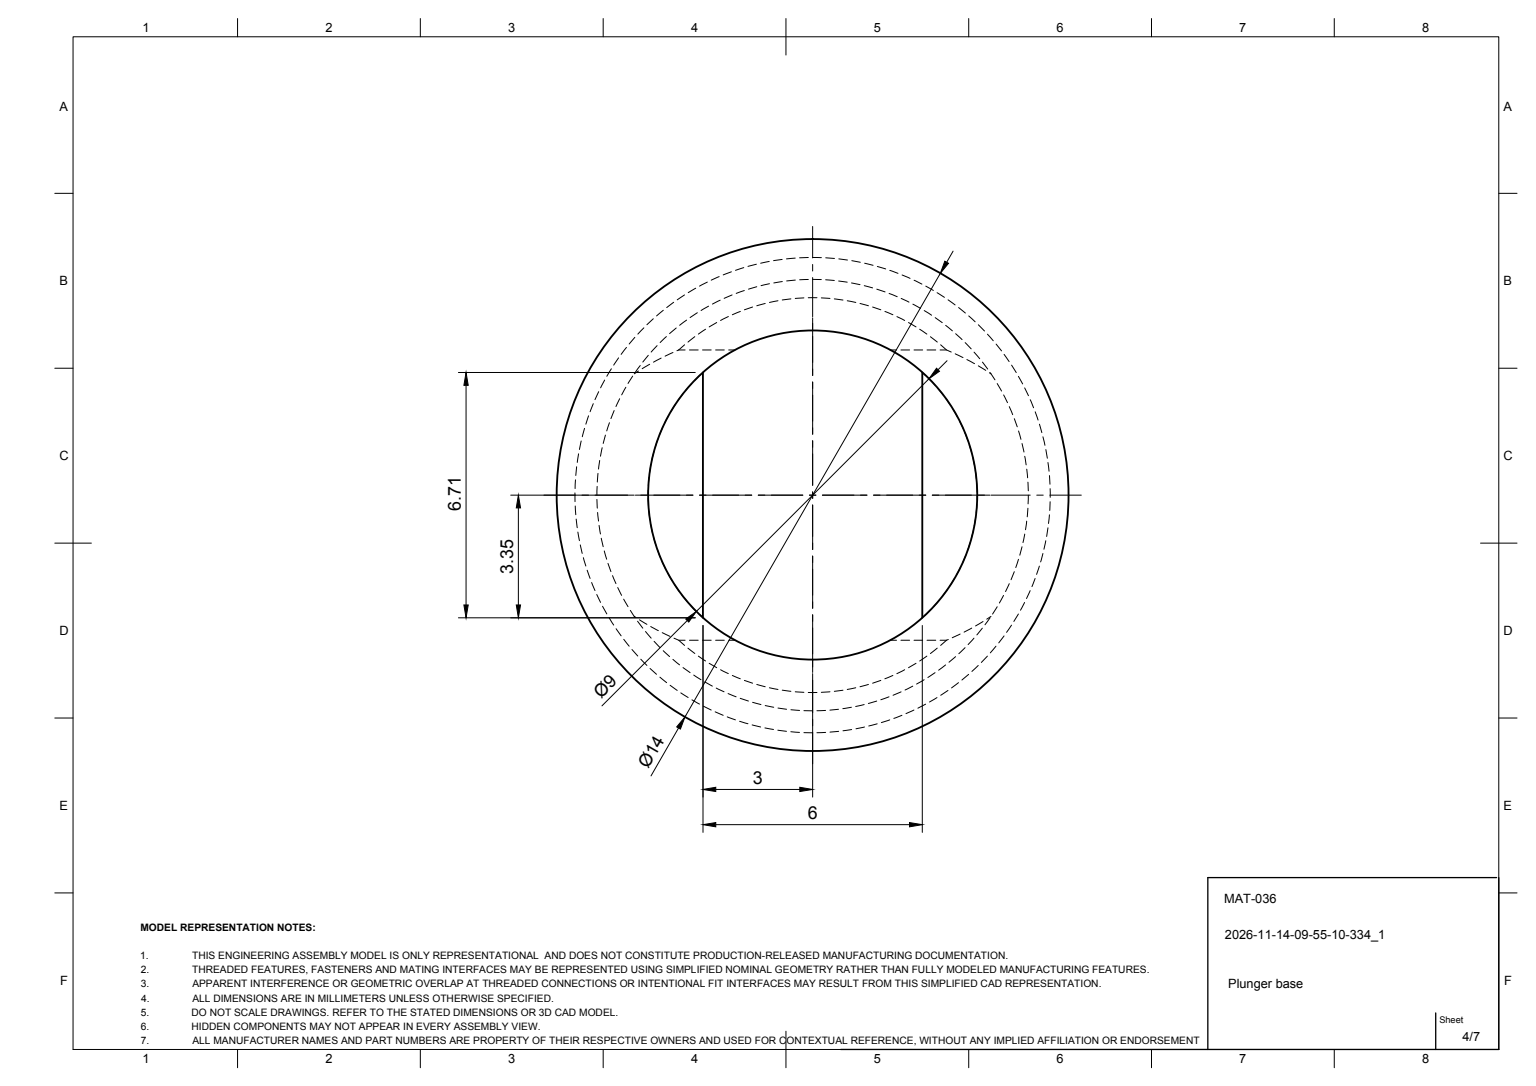
ISO-10303-21;
HEADER;
/* Generated by software containing ST-Developer
 * from STEP Tools, Inc. (www.steptools.com) 
 */

FILE_DESCRIPTION(
/* description */ (''),
/* implementation_level */ '2;1');

FILE_NAME(
/* name */ 'Plunger base.step',
/* time_stamp */ '2026-11-14T09:55:16-08:00',
/* author */ (''),
/* organization */ (''),
/* preprocessor_version */ 'ST-DEVELOPER v20.2',
/* originating_system */ 'Autodesk Translation Framework v15.17.0.0',
/* authorisation */ '');

FILE_SCHEMA (('AUTOMOTIVE_DESIGN { 1 0 10303 214 3 1 1 }'));
ENDSEC;

DATA;
#10=MECHANICAL_DESIGN_GEOMETRIC_PRESENTATION_REPRESENTATION('',(#57,#58,#59),#170250);
#40=OPEN_SHELL('',(#71352));
#41=OPEN_SHELL('',(#71353));
#42=SHELL_BASED_SURFACE_MODEL('Body2',(#40));
#43=SHELL_BASED_SURFACE_MODEL('Body3',(#41));
#45=SHAPE_REPRESENTATION_RELATIONSHIP('SRR','None',#170277,#51);
#51=ADVANCED_BREP_SHAPE_REPRESENTATION('',(#65),#170245);
#57=STYLED_ITEM('',(#170314),#65);
#58=STYLED_ITEM('',(#170314),#42);
#59=STYLED_ITEM('',(#170314),#43);
#65=MANIFOLD_SOLID_BREP('Body1',#71399);
#74=FACE_BOUND('',#15862,.T.);
#75=FACE_BOUND('',#15864,.T.);
#90=PLANE('',#77665);
#91=PLANE('',#77666);
#92=PLANE('',#77667);
#93=PLANE('',#77670);
#94=PLANE('',#77672);
#95=PLANE('',#77673);
#96=PLANE('',#77674);
#97=PLANE('',#77675);
#5361=CYLINDRICAL_SURFACE('',#77642,7.);
#5362=CYLINDRICAL_SURFACE('',#77645,4.5);
#5363=CYLINDRICAL_SURFACE('',#77652,6.5);
#5364=CYLINDRICAL_SURFACE('',#77656,5.99999999999999);
#5365=CYLINDRICAL_SURFACE('',#77663,5.9);
#5366=CYLINDRICAL_SURFACE('',#77669,5.99999999999999);
#5367=CYLINDRICAL_SURFACE('',#77677,6.);
#5368=CYLINDRICAL_SURFACE('',#77679,6.);
#10585=FACE_OUTER_BOUND('',#15854,.T.);
#10586=FACE_OUTER_BOUND('',#15855,.T.);
#10587=FACE_OUTER_BOUND('',#15856,.T.);
#10588=FACE_OUTER_BOUND('',#15857,.T.);
#10589=FACE_OUTER_BOUND('',#15858,.T.);
#10590=FACE_OUTER_BOUND('',#15859,.T.);
#10591=FACE_OUTER_BOUND('',#15860,.T.);
#10592=FACE_OUTER_BOUND('',#15861,.T.);
#10593=FACE_OUTER_BOUND('',#15863,.T.);
#10594=FACE_OUTER_BOUND('',#15865,.T.);
#10595=FACE_OUTER_BOUND('',#15866,.T.);
#10596=FACE_OUTER_BOUND('',#15867,.T.);
#10597=FACE_OUTER_BOUND('',#15868,.T.);
#10598=FACE_OUTER_BOUND('',#15869,.T.);
#10599=FACE_OUTER_BOUND('',#15870,.T.);
#10600=FACE_OUTER_BOUND('',#15871,.T.);
#10601=FACE_OUTER_BOUND('',#15872,.T.);
#10602=FACE_OUTER_BOUND('',#15873,.T.);
#10603=FACE_OUTER_BOUND('',#15874,.T.);
#15854=EDGE_LOOP('',(#65684,#65685,#65686,#65687));
#15855=EDGE_LOOP('',(#65688,#65689,#65690,#65691,#65692,#65693,#65694,#65695,
#65696,#65697,#65698,#65699,#65700,#65701,#65702,#65703));
#15856=EDGE_LOOP('',(#65704,#65705,#65706,#65707,#65708));
#15857=EDGE_LOOP('',(#65709,#65710,#65711,#65712,#65713,#65714,#65715,#65716));
#15858=EDGE_LOOP('',(#65717,#65718,#65719,#65720,#65721));
#15859=EDGE_LOOP('',(#65722,#65723,#65724,#65725));
#15860=EDGE_LOOP('',(#65726,#65727,#65728,#65729,#65730,#65731,#65732,#65733));
#15861=EDGE_LOOP('',(#65734));
#15862=EDGE_LOOP('',(#65735));
#15863=EDGE_LOOP('',(#65736));
#15864=EDGE_LOOP('',(#65737));
#15865=EDGE_LOOP('',(#65738,#65739,#65740,#65741));
#15866=EDGE_LOOP('',(#65742,#65743,#65744,#65745,#65746,#65747,#65748,#65749,
#65750));
#15867=EDGE_LOOP('',(#65751,#65752,#65753,#65754));
#15868=EDGE_LOOP('',(#65755,#65756,#65757,#65758));
#15869=EDGE_LOOP('',(#65759,#65760));
#15870=EDGE_LOOP('',(#65761,#65762,#65763));
#15871=EDGE_LOOP('',(#65764,#65765,#65766,#65767));
#15872=EDGE_LOOP('',(#65768,#65769,#65770,#65771));
#15873=EDGE_LOOP('',(#65772,#65773,#65774));
#15874=EDGE_LOOP('',(#65775,#65776,#65777));
#20991=CIRCLE('',#77643,7.);
#20992=CIRCLE('',#77644,7.);
#20993=CIRCLE('',#77646,4.5);
#20994=CIRCLE('',#77647,4.5);
#20995=CIRCLE('',#77648,4.5);
#20996=CIRCLE('',#77649,4.5);
#20997=CIRCLE('',#77650,4.5);
#20998=CIRCLE('',#77651,4.5);
#20999=CIRCLE('',#77653,6.5);
#21000=CIRCLE('',#77654,6.5);
#21001=CIRCLE('',#77655,6.5);
#21002=CIRCLE('',#77657,5.99999999999999);
#21003=CIRCLE('',#77659,5.9);
#21004=CIRCLE('',#77661,5.39999999999997);
#21005=CIRCLE('',#77662,5.9);
#21006=CIRCLE('',#77664,5.9);
#21007=CIRCLE('',#77668,5.99999999999999);
#21008=CIRCLE('',#77671,5.4);
#21009=CIRCLE('',#77678,6.);
#21010=CIRCLE('',#77680,6.);
#24303=B_SPLINE_CURVE_WITH_KNOTS('',3,(#168059,#168060,#168061,#168062),
 .UNSPECIFIED.,.F.,.F.,(4,4),(1.09971404256795,1.21244876000028),
 .UNSPECIFIED.);
#24304=B_SPLINE_CURVE_WITH_KNOTS('',3,(#168066,#168067,#168068,#168069),
 .UNSPECIFIED.,.F.,.F.,(4,4),(1.65787808514986,1.77061280261397),
 .UNSPECIFIED.);
#24305=B_SPLINE_CURVE_WITH_KNOTS('',3,(#168082,#168083,#168084,#168085),
 .UNSPECIFIED.,.F.,.F.,(4,4),(2.53487746522254,2.64761218276488),
 .UNSPECIFIED.);
#24306=B_SPLINE_CURVE_WITH_KNOTS('',3,(#168089,#168090,#168091,#168092),
 .UNSPECIFIED.,.F.,.F.,(4,4),(-2.64761218272936,-2.53487746528608),
 .UNSPECIFIED.);
#24307=B_SPLINE_CURVE_WITH_KNOTS('',3,(#168105,#168106,#168107,#168108,
#168109,#168110,#168111,#168112,#168113,#168114,#168115,#168116,#168117,
#168118),.UNSPECIFIED.,.F.,.F.,(4,2,2,2,2,2,4),(-3.61371859075551,-3.49762439616657,
-3.37604729441128,-3.254470192656,-3.13289309090071,-3.01131598914542,-2.89522179460579),
 .UNSPECIFIED.);
#24308=B_SPLINE_CURVE_WITH_KNOTS('',3,(#168120,#168121,#168122,#168123,
#168124,#168125),.UNSPECIFIED.,.F.,.F.,(4,2,4),(-0.505642410187432,-0.432426511837419,
-0.363335115211808),.UNSPECIFIED.);
#24309=B_SPLINE_CURVE_WITH_KNOTS('',3,(#168130,#168131,#168132,#168133,
#168134,#168135),.UNSPECIFIED.,.F.,.F.,(4,2,4),(-1.44175006264287,-1.37265866586429,
-1.29944276755287),.UNSPECIFIED.);
#24310=B_SPLINE_CURVE_WITH_KNOTS('',3,(#168144,#168145,#168146,#168147,
#168148,#168149),.UNSPECIFIED.,.F.,.F.,(4,2,4),(1.30070391833721,1.41679560118766,
1.44118086035152),.UNSPECIFIED.);
#24311=B_SPLINE_CURVE_WITH_KNOTS('',3,(#168155,#168156,#168157,#168158,
#168159,#168160,#168161,#168162),.UNSPECIFIED.,.F.,.F.,(4,2,2,4),(-3.254470192656,
-3.13289309090071,-3.01131598914542,-2.89522179462825),.UNSPECIFIED.);
#24312=B_SPLINE_CURVE_WITH_KNOTS('',3,(#168164,#168165,#168166,#168167,
#168168,#168169,#168170,#168171),.UNSPECIFIED.,.F.,.F.,(4,2,2,4),(-3.61371859064193,
-3.49762439616657,-3.37604729441128,-3.254470192656),.UNSPECIFIED.);
#24313=B_SPLINE_CURVE_WITH_KNOTS('',3,(#168180,#168181,#168182,#168183,
#168184,#168185),.UNSPECIFIED.,.F.,.F.,(4,2,4),(0.36333511511172,0.43242651183742,
0.505642410213935),.UNSPECIFIED.);
#24314=B_SPLINE_CURVE_WITH_KNOTS('',3,(#168200,#168201,#168202,#168203,
#168204,#168205,#168206,#168207,#168208,#168209,#168210,#168211,#168212,
#168213,#168214,#168215,#168216,#168217,#168218,#168219,#168220,#168221,
#168222,#168223,#168224,#168225,#168226,#168227,#168228,#168229,#168230,
#168231,#168232,#168233,#168234,#168235,#168236,#168237,#168238,#168239,
#168240,#168241,#168242),.UNSPECIFIED.,.F.,.F.,(4,3,3,3,3,3,3,3,3,3,3,3,
3,3,4),(0.499343871841187,0.549093604143059,0.599465023228859,0.62450790388089,
0.689718293200921,0.749671935920592,0.758683676198281,0.765317439925555,
0.780962943930518,0.812253951940444,0.874835967960296,0.890796391310028,
0.906126975970222,0.959821021734887,1.),.UNSPECIFIED.);
#24315=B_SPLINE_CURVE_WITH_KNOTS('',3,(#168243,#168244,#168245,#168246,
#168247,#168248,#168249,#168250,#168251,#168252,#168253,#168254,#168255,
#168256,#168257,#168258,#168259,#168260,#168261,#168262,#168263,#168264,
#168265,#168266,#168267,#168268,#168269,#168270,#168271,#168272,#168273,
#168274,#168275,#168276,#168277,#168278,#168279,#168280,#168281,#168282,
#168283,#168284,#168285,#168286,#168287,#168288),.UNSPECIFIED.,.F.,.F.,
(4,3,3,3,3,3,3,3,3,3,3,3,3,3,3,4),(0.,0.0539371583026244,0.106650915602551,
0.124835967960296,0.140821762748041,0.15604495995037,0.214914746357673,
0.249671935920592,0.255809368181488,0.25747418391811,0.265276431915629,
0.280880927910666,0.312089919900741,0.374507903880889,0.438618517613949,
0.499343871841187),.UNSPECIFIED.);
#24316=B_SPLINE_CURVE_WITH_KNOTS('',3,(#168292,#168293,#168294,#168295,
#168296,#168297,#168298,#168299,#168300,#168301,#168302,#168303,#168304,
#168305,#168306,#168307,#168308,#168309,#168310,#168311,#168312,#168313,
#168314,#168315,#168316,#168317,#168318,#168319,#168320,#168321,#168322,
#168323,#168324,#168325,#168326,#168327,#168328,#168329,#168330,#168331,
#168332,#168333,#168334),.UNSPECIFIED.,.F.,.F.,(4,3,3,3,3,3,3,3,3,3,3,3,
3,3,4),(0.499343871841254,0.54909365836049,0.599465134382744,0.62450790388094,
0.689718289747475,0.749671935920627,0.758683679203924,0.765317439925588,
0.780962943930549,0.812253951940471,0.874835967960314,0.890796399632331,
0.906126975970235,0.959821023994028,1.),.UNSPECIFIED.);
#24317=B_SPLINE_CURVE_WITH_KNOTS('',3,(#168336,#168337,#168338,#168339,
#168340,#168341,#168342,#168343,#168344,#168345,#168346,#168347,#168348,
#168349,#168350,#168351,#168352,#168353,#168354,#168355,#168356,#168357,
#168358,#168359,#168360,#168361,#168362,#168363,#168364,#168365,#168366,
#168367,#168368,#168369,#168370,#168371,#168372,#168373,#168374,#168375,
#168376,#168377,#168378,#168379,#168380,#168381),.UNSPECIFIED.,.F.,.F.,
(4,3,3,3,3,3,3,3,3,3,3,3,3,3,3,4),(0.,0.0539371583336762,0.10665091566333,
0.124835967960314,0.140821762714439,0.156044959950392,0.214914746428806,
0.249671935920627,0.255809368181394,0.257474183918147,0.265276431915666,
0.280880927910705,0.312089919900784,0.37450790388094,0.438618517375844,
0.499343871841254),.UNSPECIFIED.);
#26394=LINE('',#168050,#28482);
#26395=LINE('',#168057,#28483);
#26396=LINE('',#168071,#28484);
#26397=LINE('',#168075,#28485);
#26398=LINE('',#168080,#28486);
#26399=LINE('',#168093,#28487);
#26400=LINE('',#168100,#28488);
#26401=LINE('',#168126,#28489);
#26402=LINE('',#168129,#28490);
#26403=LINE('',#168138,#28491);
#26404=LINE('',#168153,#28492);
#26405=LINE('',#168176,#28493);
#26406=LINE('',#168179,#28494);
#26407=LINE('',#168186,#28495);
#26408=LINE('',#168190,#28496);
#28482=VECTOR('',#92146,7.);
#28483=VECTOR('',#92153,1000.);
#28484=VECTOR('',#92156,1000.);
#28485=VECTOR('',#92159,4.5);
#28486=VECTOR('',#92164,1000.);
#28487=VECTOR('',#92167,1000.);
#28488=VECTOR('',#92174,6.5);
#28489=VECTOR('',#92179,1000.);
#28490=VECTOR('',#92182,1000.);
#28491=VECTOR('',#92185,5.9);
#28492=VECTOR('',#92196,5.9);
#28493=VECTOR('',#92207,1000.);
#28494=VECTOR('',#92210,1000.);
#28495=VECTOR('',#92211,1000.);
#28496=VECTOR('',#92218,1000.);
#33854=VERTEX_POINT('',#168047);
#33855=VERTEX_POINT('',#168049);
#33856=VERTEX_POINT('',#168053);
#33857=VERTEX_POINT('',#168054);
#33858=VERTEX_POINT('',#168056);
#33859=VERTEX_POINT('',#168058);
#33860=VERTEX_POINT('',#168063);
#33861=VERTEX_POINT('',#168065);
#33862=VERTEX_POINT('',#168070);
#33863=VERTEX_POINT('',#168072);
#33864=VERTEX_POINT('',#168074);
#33865=VERTEX_POINT('',#168077);
#33866=VERTEX_POINT('',#168079);
#33867=VERTEX_POINT('',#168081);
#33868=VERTEX_POINT('',#168086);
#33869=VERTEX_POINT('',#168088);
#33870=VERTEX_POINT('',#168095);
#33871=VERTEX_POINT('',#168096);
#33872=VERTEX_POINT('',#168099);
#33873=VERTEX_POINT('',#168103);
#33874=VERTEX_POINT('',#168104);
#33875=VERTEX_POINT('',#168119);
#33876=VERTEX_POINT('',#168128);
#33877=VERTEX_POINT('',#168137);
#33878=VERTEX_POINT('',#168141);
#33879=VERTEX_POINT('',#168143);
#33880=VERTEX_POINT('',#168152);
#33881=VERTEX_POINT('',#168154);
#33882=VERTEX_POINT('',#168178);
#33883=VERTEX_POINT('',#168196);
#33884=VERTEX_POINT('',#168197);
#33885=VERTEX_POINT('',#168199);
#33886=VERTEX_POINT('',#168290);
#33887=VERTEX_POINT('',#168291);
#33888=VERTEX_POINT('',#168335);
#44483=EDGE_CURVE('',#33854,#33854,#20991,.T.);
#44484=EDGE_CURVE('',#33854,#33855,#26394,.T.);
#44485=EDGE_CURVE('',#33855,#33855,#20992,.T.);
#44486=EDGE_CURVE('',#33856,#33857,#20993,.T.);
#44487=EDGE_CURVE('',#33857,#33858,#26395,.T.);
#44488=EDGE_CURVE('',#33858,#33859,#24303,.T.);
#44489=EDGE_CURVE('',#33859,#33860,#20994,.T.);
#44490=EDGE_CURVE('',#33860,#33861,#24304,.T.);
#44491=EDGE_CURVE('',#33861,#33862,#26396,.T.);
#44492=EDGE_CURVE('',#33862,#33863,#20995,.T.);
#44493=EDGE_CURVE('',#33863,#33864,#26397,.T.);
#44494=EDGE_CURVE('',#33864,#33864,#20996,.T.);
#44495=EDGE_CURVE('',#33863,#33865,#20997,.T.);
#44496=EDGE_CURVE('',#33865,#33866,#26398,.T.);
#44497=EDGE_CURVE('',#33866,#33867,#24305,.T.);
#44498=EDGE_CURVE('',#33867,#33868,#20998,.T.);
#44499=EDGE_CURVE('',#33868,#33869,#24306,.T.);
#44500=EDGE_CURVE('',#33869,#33856,#26399,.T.);
#44501=EDGE_CURVE('',#33870,#33871,#20999,.T.);
#44502=EDGE_CURVE('',#33871,#33870,#21000,.T.);
#44503=EDGE_CURVE('',#33871,#33872,#26400,.T.);
#44504=EDGE_CURVE('',#33872,#33872,#21001,.T.);
#44505=EDGE_CURVE('',#33873,#33874,#24307,.T.);
#44506=EDGE_CURVE('',#33874,#33875,#24308,.T.);
#44507=EDGE_CURVE('',#33859,#33875,#26401,.T.);
#44508=EDGE_CURVE('',#33858,#33869,#21002,.T.);
#44509=EDGE_CURVE('',#33868,#33876,#26402,.T.);
#44510=EDGE_CURVE('',#33876,#33873,#24309,.T.);
#44511=EDGE_CURVE('',#33870,#33877,#26403,.T.);
#44512=EDGE_CURVE('',#33877,#33877,#21003,.T.);
#44513=EDGE_CURVE('',#33878,#33876,#21004,.T.);
#44514=EDGE_CURVE('',#33879,#33878,#24310,.T.);
#44515=EDGE_CURVE('',#33873,#33879,#21005,.T.);
#44516=EDGE_CURVE('',#33877,#33880,#26404,.T.);
#44517=EDGE_CURVE('',#33881,#33880,#24311,.F.);
#44518=EDGE_CURVE('',#33874,#33881,#21006,.T.);
#44519=EDGE_CURVE('',#33880,#33879,#24312,.F.);
#44520=EDGE_CURVE('',#33861,#33866,#21007,.T.);
#44521=EDGE_CURVE('',#33865,#33862,#26405,.T.);
#44522=EDGE_CURVE('',#33860,#33882,#26406,.T.);
#44523=EDGE_CURVE('',#33882,#33881,#24313,.T.);
#44524=EDGE_CURVE('',#33878,#33867,#26407,.T.);
#44525=EDGE_CURVE('',#33875,#33882,#21008,.T.);
#44526=EDGE_CURVE('',#33857,#33856,#26408,.T.);
#44527=EDGE_CURVE('',#33883,#33884,#21009,.T.);
#44528=EDGE_CURVE('',#33885,#33883,#24314,.T.);
#44529=EDGE_CURVE('',#33884,#33885,#24315,.T.);
#44530=EDGE_CURVE('',#33886,#33887,#24316,.T.);
#44531=EDGE_CURVE('',#33888,#33886,#24317,.T.);
#44532=EDGE_CURVE('',#33887,#33888,#21010,.T.);
#65684=ORIENTED_EDGE('',*,*,#44483,.F.);
#65685=ORIENTED_EDGE('',*,*,#44484,.T.);
#65686=ORIENTED_EDGE('',*,*,#44485,.F.);
#65687=ORIENTED_EDGE('',*,*,#44484,.F.);
#65688=ORIENTED_EDGE('',*,*,#44486,.T.);
#65689=ORIENTED_EDGE('',*,*,#44487,.T.);
#65690=ORIENTED_EDGE('',*,*,#44488,.T.);
#65691=ORIENTED_EDGE('',*,*,#44489,.T.);
#65692=ORIENTED_EDGE('',*,*,#44490,.T.);
#65693=ORIENTED_EDGE('',*,*,#44491,.T.);
#65694=ORIENTED_EDGE('',*,*,#44492,.T.);
#65695=ORIENTED_EDGE('',*,*,#44493,.T.);
#65696=ORIENTED_EDGE('',*,*,#44494,.F.);
#65697=ORIENTED_EDGE('',*,*,#44493,.F.);
#65698=ORIENTED_EDGE('',*,*,#44495,.T.);
#65699=ORIENTED_EDGE('',*,*,#44496,.T.);
#65700=ORIENTED_EDGE('',*,*,#44497,.T.);
#65701=ORIENTED_EDGE('',*,*,#44498,.T.);
#65702=ORIENTED_EDGE('',*,*,#44499,.T.);
#65703=ORIENTED_EDGE('',*,*,#44500,.T.);
#65704=ORIENTED_EDGE('',*,*,#44501,.F.);
#65705=ORIENTED_EDGE('',*,*,#44502,.F.);
#65706=ORIENTED_EDGE('',*,*,#44503,.T.);
#65707=ORIENTED_EDGE('',*,*,#44504,.T.);
#65708=ORIENTED_EDGE('',*,*,#44503,.F.);
#65709=ORIENTED_EDGE('',*,*,#44505,.T.);
#65710=ORIENTED_EDGE('',*,*,#44506,.T.);
#65711=ORIENTED_EDGE('',*,*,#44507,.F.);
#65712=ORIENTED_EDGE('',*,*,#44488,.F.);
#65713=ORIENTED_EDGE('',*,*,#44508,.T.);
#65714=ORIENTED_EDGE('',*,*,#44499,.F.);
#65715=ORIENTED_EDGE('',*,*,#44509,.T.);
#65716=ORIENTED_EDGE('',*,*,#44510,.T.);
#65717=ORIENTED_EDGE('',*,*,#44501,.T.);
#65718=ORIENTED_EDGE('',*,*,#44502,.T.);
#65719=ORIENTED_EDGE('',*,*,#44511,.T.);
#65720=ORIENTED_EDGE('',*,*,#44512,.F.);
#65721=ORIENTED_EDGE('',*,*,#44511,.F.);
#65722=ORIENTED_EDGE('',*,*,#44513,.F.);
#65723=ORIENTED_EDGE('',*,*,#44514,.F.);
#65724=ORIENTED_EDGE('',*,*,#44515,.F.);
#65725=ORIENTED_EDGE('',*,*,#44510,.F.);
#65726=ORIENTED_EDGE('',*,*,#44512,.T.);
#65727=ORIENTED_EDGE('',*,*,#44516,.T.);
#65728=ORIENTED_EDGE('',*,*,#44517,.F.);
#65729=ORIENTED_EDGE('',*,*,#44518,.F.);
#65730=ORIENTED_EDGE('',*,*,#44505,.F.);
#65731=ORIENTED_EDGE('',*,*,#44515,.T.);
#65732=ORIENTED_EDGE('',*,*,#44519,.F.);
#65733=ORIENTED_EDGE('',*,*,#44516,.F.);
#65734=ORIENTED_EDGE('',*,*,#44485,.T.);
#65735=ORIENTED_EDGE('',*,*,#44494,.T.);
#65736=ORIENTED_EDGE('',*,*,#44483,.T.);
#65737=ORIENTED_EDGE('',*,*,#44504,.F.);
#65738=ORIENTED_EDGE('',*,*,#44520,.T.);
#65739=ORIENTED_EDGE('',*,*,#44496,.F.);
#65740=ORIENTED_EDGE('',*,*,#44521,.T.);
#65741=ORIENTED_EDGE('',*,*,#44491,.F.);
#65742=ORIENTED_EDGE('',*,*,#44520,.F.);
#65743=ORIENTED_EDGE('',*,*,#44490,.F.);
#65744=ORIENTED_EDGE('',*,*,#44522,.T.);
#65745=ORIENTED_EDGE('',*,*,#44523,.T.);
#65746=ORIENTED_EDGE('',*,*,#44517,.T.);
#65747=ORIENTED_EDGE('',*,*,#44519,.T.);
#65748=ORIENTED_EDGE('',*,*,#44514,.T.);
#65749=ORIENTED_EDGE('',*,*,#44524,.T.);
#65750=ORIENTED_EDGE('',*,*,#44497,.F.);
#65751=ORIENTED_EDGE('',*,*,#44507,.T.);
#65752=ORIENTED_EDGE('',*,*,#44525,.T.);
#65753=ORIENTED_EDGE('',*,*,#44522,.F.);
#65754=ORIENTED_EDGE('',*,*,#44489,.F.);
#65755=ORIENTED_EDGE('',*,*,#44508,.F.);
#65756=ORIENTED_EDGE('',*,*,#44487,.F.);
#65757=ORIENTED_EDGE('',*,*,#44526,.T.);
#65758=ORIENTED_EDGE('',*,*,#44500,.F.);
#65759=ORIENTED_EDGE('',*,*,#44526,.F.);
#65760=ORIENTED_EDGE('',*,*,#44486,.F.);
#65761=ORIENTED_EDGE('',*,*,#44521,.F.);
#65762=ORIENTED_EDGE('',*,*,#44495,.F.);
#65763=ORIENTED_EDGE('',*,*,#44492,.F.);
#65764=ORIENTED_EDGE('',*,*,#44524,.F.);
#65765=ORIENTED_EDGE('',*,*,#44513,.T.);
#65766=ORIENTED_EDGE('',*,*,#44509,.F.);
#65767=ORIENTED_EDGE('',*,*,#44498,.F.);
#65768=ORIENTED_EDGE('',*,*,#44506,.F.);
#65769=ORIENTED_EDGE('',*,*,#44518,.T.);
#65770=ORIENTED_EDGE('',*,*,#44523,.F.);
#65771=ORIENTED_EDGE('',*,*,#44525,.F.);
#65772=ORIENTED_EDGE('',*,*,#44527,.F.);
#65773=ORIENTED_EDGE('',*,*,#44528,.F.);
#65774=ORIENTED_EDGE('',*,*,#44529,.F.);
#65775=ORIENTED_EDGE('',*,*,#44530,.F.);
#65776=ORIENTED_EDGE('',*,*,#44531,.F.);
#65777=ORIENTED_EDGE('',*,*,#44532,.F.);
#66124=CONICAL_SURFACE('',#77658,5.9,0.785398163397448);
#66125=CONICAL_SURFACE('',#77660,5.40000000000002,0.785398163397455);
#66126=CONICAL_SURFACE('',#77676,5.4,0.785398163397447);
#71335=ADVANCED_FACE('',(#10585),#5361,.T.);
#71336=ADVANCED_FACE('',(#10586),#5362,.F.);
#71337=ADVANCED_FACE('',(#10587),#5363,.T.);
#71338=ADVANCED_FACE('',(#10588),#5364,.F.);
#71339=ADVANCED_FACE('',(#10589),#66124,.T.);
#71340=ADVANCED_FACE('',(#10590),#66125,.T.);
#71341=ADVANCED_FACE('',(#10591),#5365,.T.);
#71342=ADVANCED_FACE('',(#10592,#74),#90,.T.);
#71343=ADVANCED_FACE('',(#10593,#75),#91,.F.);
#71344=ADVANCED_FACE('',(#10594),#92,.T.);
#71345=ADVANCED_FACE('',(#10595),#5366,.F.);
#71346=ADVANCED_FACE('',(#10596),#93,.T.);
#71347=ADVANCED_FACE('',(#10597),#94,.T.);
#71348=ADVANCED_FACE('',(#10598),#95,.T.);
#71349=ADVANCED_FACE('',(#10599),#96,.T.);
#71350=ADVANCED_FACE('',(#10600),#97,.T.);
#71351=ADVANCED_FACE('',(#10601),#66126,.T.);
#71352=ADVANCED_FACE('',(#10602),#5367,.T.);
#71353=ADVANCED_FACE('',(#10603),#5368,.T.);
#71399=CLOSED_SHELL('',(#71335,#71336,#71337,#71338,#71339,#71340,#71341,
#71342,#71343,#71344,#71345,#71346,#71347,#71348,#71349,#71350,#71351));
#77641=AXIS2_PLACEMENT_3D('',#168045,#92140,#92141);
#77642=AXIS2_PLACEMENT_3D('',#168046,#92142,#92143);
#77643=AXIS2_PLACEMENT_3D('',#168048,#92144,#92145);
#77644=AXIS2_PLACEMENT_3D('',#168051,#92147,#92148);
#77645=AXIS2_PLACEMENT_3D('',#168052,#92149,#92150);
#77646=AXIS2_PLACEMENT_3D('',#168055,#92151,#92152);
#77647=AXIS2_PLACEMENT_3D('',#168064,#92154,#92155);
#77648=AXIS2_PLACEMENT_3D('',#168073,#92157,#92158);
#77649=AXIS2_PLACEMENT_3D('',#168076,#92160,#92161);
#77650=AXIS2_PLACEMENT_3D('',#168078,#92162,#92163);
#77651=AXIS2_PLACEMENT_3D('',#168087,#92165,#92166);
#77652=AXIS2_PLACEMENT_3D('',#168094,#92168,#92169);
#77653=AXIS2_PLACEMENT_3D('',#168097,#92170,#92171);
#77654=AXIS2_PLACEMENT_3D('',#168098,#92172,#92173);
#77655=AXIS2_PLACEMENT_3D('',#168101,#92175,#92176);
#77656=AXIS2_PLACEMENT_3D('',#168102,#92177,#92178);
#77657=AXIS2_PLACEMENT_3D('',#168127,#92180,#92181);
#77658=AXIS2_PLACEMENT_3D('',#168136,#92183,#92184);
#77659=AXIS2_PLACEMENT_3D('',#168139,#92186,#92187);
#77660=AXIS2_PLACEMENT_3D('',#168140,#92188,#92189);
#77661=AXIS2_PLACEMENT_3D('',#168142,#92190,#92191);
#77662=AXIS2_PLACEMENT_3D('',#168150,#92192,#92193);
#77663=AXIS2_PLACEMENT_3D('',#168151,#92194,#92195);
#77664=AXIS2_PLACEMENT_3D('',#168163,#92197,#92198);
#77665=AXIS2_PLACEMENT_3D('',#168172,#92199,#92200);
#77666=AXIS2_PLACEMENT_3D('',#168173,#92201,#92202);
#77667=AXIS2_PLACEMENT_3D('',#168174,#92203,#92204);
#77668=AXIS2_PLACEMENT_3D('',#168175,#92205,#92206);
#77669=AXIS2_PLACEMENT_3D('',#168177,#92208,#92209);
#77670=AXIS2_PLACEMENT_3D('',#168187,#92212,#92213);
#77671=AXIS2_PLACEMENT_3D('',#168188,#92214,#92215);
#77672=AXIS2_PLACEMENT_3D('',#168189,#92216,#92217);
#77673=AXIS2_PLACEMENT_3D('',#168191,#92219,#92220);
#77674=AXIS2_PLACEMENT_3D('',#168192,#92221,#92222);
#77675=AXIS2_PLACEMENT_3D('',#168193,#92223,#92224);
#77676=AXIS2_PLACEMENT_3D('',#168194,#92225,#92226);
#77677=AXIS2_PLACEMENT_3D('',#168195,#92227,#92228);
#77678=AXIS2_PLACEMENT_3D('',#168198,#92229,#92230);
#77679=AXIS2_PLACEMENT_3D('',#168289,#92231,#92232);
#77680=AXIS2_PLACEMENT_3D('',#168382,#92233,#92234);
#92140=DIRECTION('axis',(0.,0.,1.));
#92141=DIRECTION('refdir',(1.,0.,0.));
#92142=DIRECTION('center_axis',(5.28813965849088E-17,1.,5.28813965824263E-17));
#92143=DIRECTION('ref_axis',(-1.,5.28813965849088E-17,-4.79793613002828E-34));
#92144=DIRECTION('center_axis',(5.28813965849088E-17,1.,5.28813965824263E-17));
#92145=DIRECTION('ref_axis',(-1.,5.28813965849088E-17,-4.79793613002828E-34));
#92146=DIRECTION('',(-5.28813965849088E-17,-1.,-5.28813965824263E-17));
#92147=DIRECTION('center_axis',(-5.28813965849088E-17,-1.,-5.28813965824263E-17));
#92148=DIRECTION('ref_axis',(-1.,5.28813965849088E-17,-4.79793613002828E-34));
#92149=DIRECTION('center_axis',(0.,-1.,0.));
#92150=DIRECTION('ref_axis',(0.,0.,-1.));
#92151=DIRECTION('center_axis',(0.,1.,0.));
#92152=DIRECTION('ref_axis',(0.,0.,-1.));
#92153=DIRECTION('',(0.,1.,0.));
#92154=DIRECTION('center_axis',(0.,1.,0.));
#92155=DIRECTION('ref_axis',(0.,0.,-1.));
#92156=DIRECTION('',(0.,-1.,0.));
#92157=DIRECTION('center_axis',(0.,1.,0.));
#92158=DIRECTION('ref_axis',(1.77635683940025E-15,0.,-1.));
#92159=DIRECTION('',(0.,-1.,0.));
#92160=DIRECTION('center_axis',(0.,1.,0.));
#92161=DIRECTION('ref_axis',(0.,0.,-1.));
#92162=DIRECTION('center_axis',(0.,1.,0.));
#92163=DIRECTION('ref_axis',(1.77635683940025E-15,0.,-1.));
#92164=DIRECTION('',(-2.63231840778213E-15,1.,2.63231840765855E-15));
#92165=DIRECTION('center_axis',(-2.63231840778213E-15,1.,2.63231840765855E-15));
#92166=DIRECTION('ref_axis',(1.,2.63231840778213E-15,-1.74102415060709E-31));
#92167=DIRECTION('',(2.63231840778213E-15,-1.,-2.63231840765855E-15));
#92168=DIRECTION('center_axis',(0.,1.,1.66800334228539E-17));
#92169=DIRECTION('ref_axis',(0.,-1.66800334228539E-17,1.));
#92170=DIRECTION('center_axis',(0.,1.,1.47010464065831E-16));
#92171=DIRECTION('ref_axis',(0.,1.47010464065831E-16,-1.));
#92172=DIRECTION('center_axis',(0.,1.,1.47010464065831E-16));
#92173=DIRECTION('ref_axis',(0.,1.47010464065831E-16,-1.));
#92174=DIRECTION('',(0.,-1.,-1.66800334228539E-17));
#92175=DIRECTION('center_axis',(0.,1.,1.66800334228539E-17));
#92176=DIRECTION('ref_axis',(0.,-1.66800334228539E-17,1.));
#92177=DIRECTION('center_axis',(-2.93166199061116E-26,2.06514699531572E-15,
1.));
#92178=DIRECTION('ref_axis',(-1.21086259326173E-42,-1.,2.06514699531572E-15));
#92179=DIRECTION('',(0.,0.,-1.));
#92180=DIRECTION('center_axis',(-2.93166199061116E-26,2.06514699531572E-15,
1.));
#92181=DIRECTION('ref_axis',(9.08146939547479E-43,-1.,2.06514699531572E-15));
#92182=DIRECTION('',(2.93166199061116E-26,-2.06514699531572E-15,-1.));
#92183=DIRECTION('center_axis',(0.,-1.,-1.47010464065831E-16));
#92184=DIRECTION('ref_axis',(0.,1.47010464065831E-16,-1.));
#92185=DIRECTION('',(8.65956056235493E-17,0.707106781186548,-0.707106781186547));
#92186=DIRECTION('center_axis',(0.,1.,3.67526160164578E-16));
#92187=DIRECTION('ref_axis',(0.,3.67526160164578E-16,-1.));
#92188=DIRECTION('center_axis',(-8.85182572930084E-15,-1.,-4.71957425956767E-15));
#92189=DIRECTION('ref_axis',(1.,-8.85182572930084E-15,6.75072510268539E-31));
#92190=DIRECTION('center_axis',(-1.77036514757944E-15,1.,9.43914852352751E-16));
#92191=DIRECTION('ref_axis',(1.,1.77036514757944E-15,-1.48294102778218E-31));
#92192=DIRECTION('center_axis',(0.,-1.,3.67526160164578E-16));
#92193=DIRECTION('ref_axis',(0.,-3.67526160164578E-16,-1.));
#92194=DIRECTION('center_axis',(0.,-1.,3.67526160164578E-16));
#92195=DIRECTION('ref_axis',(0.,-3.67526160164578E-16,-1.));
#92196=DIRECTION('',(0.,1.,-3.67526160164578E-16));
#92197=DIRECTION('center_axis',(-1.45977385561436E-15,1.,6.6703545231173E-26));
#92198=DIRECTION('ref_axis',(1.,1.45977385561436E-15,-6.89099987452658E-43));
#92199=DIRECTION('center_axis',(0.,-1.,0.));
#92200=DIRECTION('ref_axis',(0.,0.,-1.));
#92201=DIRECTION('center_axis',(0.,-1.,0.));
#92202=DIRECTION('ref_axis',(0.,0.,-1.));
#92203=DIRECTION('center_axis',(0.,0.,-1.));
#92204=DIRECTION('ref_axis',(0.,-1.,0.));
#92205=DIRECTION('center_axis',(0.,0.,1.));
#92206=DIRECTION('ref_axis',(1.,0.,0.));
#92207=DIRECTION('',(-1.,0.,0.));
#92208=DIRECTION('center_axis',(0.,0.,1.));
#92209=DIRECTION('ref_axis',(1.,0.,0.));
#92210=DIRECTION('',(0.,0.,1.));
#92211=DIRECTION('',(0.,0.,-1.));
#92212=DIRECTION('center_axis',(0.,1.,0.));
#92213=DIRECTION('ref_axis',(1.,0.,0.));
#92214=DIRECTION('center_axis',(-1.45977385561436E-15,1.,6.6703545231173E-26));
#92215=DIRECTION('ref_axis',(1.,1.45977385561436E-15,8.88178419700125E-16));
#92216=DIRECTION('center_axis',(0.,0.,1.));
#92217=DIRECTION('ref_axis',(1.,0.,0.));
#92218=DIRECTION('',(1.,0.,0.));
#92219=DIRECTION('center_axis',(0.,-1.,0.));
#92220=DIRECTION('ref_axis',(0.,0.,-1.));
#92221=DIRECTION('center_axis',(0.,-1.,0.));
#92222=DIRECTION('ref_axis',(0.,0.,-1.));
#92223=DIRECTION('center_axis',(0.,1.,0.));
#92224=DIRECTION('ref_axis',(1.,0.,0.));
#92225=DIRECTION('center_axis',(1.45977385561436E-15,-1.,-6.6703545231173E-26));
#92226=DIRECTION('ref_axis',(-1.,-1.45977385561436E-15,2.10124025885857E-11));
#92227=DIRECTION('center_axis',(1.0383151449662E-25,-9.0044324180798E-16,
1.));
#92228=DIRECTION('ref_axis',(-3.43490264341233E-42,-1.,-9.0044324180798E-16));
#92229=DIRECTION('center_axis',(-1.0383151449662E-25,9.0044324180798E-16,
-1.));
#92230=DIRECTION('ref_axis',(-0.564905044898505,-0.825155918750037,-7.4300607041767E-16));
#92231=DIRECTION('center_axis',(-5.53768147829691E-25,4.80236395630922E-15,
1.));
#92232=DIRECTION('ref_axis',(-1.76510259964373E-41,-1.,4.80236395630923E-15));
#92233=DIRECTION('center_axis',(-1.0383151449662E-25,9.0044324180798E-16,
1.));
#92234=DIRECTION('ref_axis',(-0.564905044898511,-0.825155918750033,7.43006070417667E-16));
#168045=CARTESIAN_POINT('',(0.,0.,0.));
#168046=CARTESIAN_POINT('Origin',(-1.00994955198656E-15,1.2,8.96986209700434E-15));
#168047=CARTESIAN_POINT('',(6.99999999999999,1.7,8.13905003589241E-15));
#168048=CARTESIAN_POINT('Origin',(-9.8350885369411E-16,1.7,8.99630279529556E-15));
#168049=CARTESIAN_POINT('',(6.99999999999999,1.2,8.1126093376012E-15));
#168050=CARTESIAN_POINT('',(6.99999999999999,1.2,8.1126093376012E-15));
#168051=CARTESIAN_POINT('Origin',(-1.00994955198656E-15,1.2,8.96986209700434E-15));
#168052=CARTESIAN_POINT('Origin',(-2.75545529808154E-16,8.2,0.));
#168053=CARTESIAN_POINT('',(3.35410196653775,3.2,-2.99999999967796));
#168054=CARTESIAN_POINT('',(-3.35410196599079,3.2,-3.00000000028945));
#168055=CARTESIAN_POINT('Origin',(-2.75545529808154E-16,3.2,0.));
#168056=CARTESIAN_POINT('',(-3.35410196587205,7.72506281421231,-3.00000000013276));
#168057=CARTESIAN_POINT('',(-3.35410196573189,8.2,-3.00000000057891));
#168058=CARTESIAN_POINT('',(-3.9686269655808,8.2,-2.12132034546057));
#168059=CARTESIAN_POINT('Ctrl Pts',(-3.3541019659917,7.72506281429298,-3.00000000028843));
#168060=CARTESIAN_POINT('Ctrl Pts',(-3.58710885370055,7.8821560259217,-2.7394903802622));
#168061=CARTESIAN_POINT('Ctrl Pts',(-3.79652270311249,8.04821830647437,
-2.44329793762419));
#168062=CARTESIAN_POINT('Ctrl Pts',(-3.96862696573053,8.19999999923597,
-2.12132034518044));
#168063=CARTESIAN_POINT('',(-3.96862696601141,8.19999999948366,2.12132034465497));
#168064=CARTESIAN_POINT('Origin',(-2.75545529808154E-16,8.2,0.));
#168065=CARTESIAN_POINT('',(-3.35410196620117,7.72506281443419,3.00000000011756));
#168066=CARTESIAN_POINT('Ctrl Pts',(-3.96862696601141,8.19999999948366,
2.12132034465497));
#168067=CARTESIAN_POINT('Ctrl Pts',(-3.79654026724857,8.04823379656728,
2.44326507823699));
#168068=CARTESIAN_POINT('Ctrl Pts',(-3.58713416135787,7.88217308835326,
2.73946208540911));
#168069=CARTESIAN_POINT('Ctrl Pts',(-3.35410196617499,7.72506281441655,
3.00000000008351));
#168070=CARTESIAN_POINT('',(-3.35410196614453,3.2,3.00000000011756));
#168071=CARTESIAN_POINT('',(-3.35410196603938,8.2,3.00000000023512));
#168072=CARTESIAN_POINT('',(-8.26636589424463E-16,3.2,4.5));
#168073=CARTESIAN_POINT('Origin',(-2.75545529808154E-16,3.2,0.));
#168074=CARTESIAN_POINT('',(-8.26636589424463E-16,1.2,4.5));
#168075=CARTESIAN_POINT('',(-8.26636589424463E-16,8.2,4.5));
#168076=CARTESIAN_POINT('Origin',(-2.75545529808154E-16,1.2,0.));
#168077=CARTESIAN_POINT('',(3.35410196626425,3.20000000000001,2.9999999999837));
#168078=CARTESIAN_POINT('Origin',(-2.75545529808154E-16,3.2,0.));
#168079=CARTESIAN_POINT('',(3.35410196633334,7.7250628145233,2.99999999999999));
#168080=CARTESIAN_POINT('',(3.35410196627882,8.19999999999999,2.99999999996742));
#168081=CARTESIAN_POINT('',(3.96862696647739,8.19999999977888,2.12132034378318));
#168082=CARTESIAN_POINT('Ctrl Pts',(3.35410196629467,7.72506281449723,2.9999999999497));
#168083=CARTESIAN_POINT('Ctrl Pts',(3.58710885421097,7.88215602628645,2.73949037963858));
#168084=CARTESIAN_POINT('Ctrl Pts',(3.79652270377537,8.04821830700949,2.44329793664967));
#168085=CARTESIAN_POINT('Ctrl Pts',(3.96862696645806,8.19999999987757,2.12132034381937));
#168086=CARTESIAN_POINT('',(3.96862696629539,8.19999999973411,-2.12132034412369));
#168087=CARTESIAN_POINT('Origin',(-7.51257911368137E-16,8.2,-5.73912088018113E-15));
#168088=CARTESIAN_POINT('',(3.35410196681833,7.72506281485028,-2.99999999967796));
#168089=CARTESIAN_POINT('Ctrl Pts',(3.96862696629539,8.19999999973411,-2.12132034412369));
#168090=CARTESIAN_POINT('Ctrl Pts',(3.79654026760466,8.04823379686202,-2.44326507767448));
#168091=CARTESIAN_POINT('Ctrl Pts',(3.58713416179472,7.88217308868278,-2.73946208483092));
#168092=CARTESIAN_POINT('Ctrl Pts',(3.35410196668864,7.72506281476285,-2.99999999950923));
#168093=CARTESIAN_POINT('',(3.35410196682577,8.20000000000001,-2.99999999935591));
#168094=CARTESIAN_POINT('Origin',(0.,1.7,-3.98010209722891E-16));
#168095=CARTESIAN_POINT('',(7.9602041944578E-16,4.6,6.5));
#168096=CARTESIAN_POINT('',(-7.9602041944578E-16,4.6,-6.5));
#168097=CARTESIAN_POINT('Origin',(0.,4.6,-4.49477084187968E-16));
#168098=CARTESIAN_POINT('Origin',(0.,4.6,-4.49477084187968E-16));
#168099=CARTESIAN_POINT('',(-7.9602041944578E-16,1.7,-6.5));
#168100=CARTESIAN_POINT('',(-7.9602041944578E-16,1.7,-6.5));
#168101=CARTESIAN_POINT('Origin',(0.,1.7,-3.98010209722891E-16));
#168102=CARTESIAN_POINT('Origin',(6.07153216591882E-15,12.7,-5.92306788700001));
#168103=CARTESIAN_POINT('',(3.31662479106209,7.70000000046876,-4.87954915902201));
#168104=CARTESIAN_POINT('',(-3.31662479061361,7.70000000017128,-4.87954915911973));
#168105=CARTESIAN_POINT('Ctrl Pts',(3.31662479106319,7.7000000004695,-4.87954915902126));
#168106=CARTESIAN_POINT('Ctrl Pts',(3.02283773840257,7.50512371602168,-5.07923593138345));
#168107=CARTESIAN_POINT('Ctrl Pts',(2.69989199164368,7.32869287193907,-5.2594505282712));
#168108=CARTESIAN_POINT('Ctrl Pts',(1.99447655600236,7.02761131950198,-5.56659302751097));
#168109=CARTESIAN_POINT('Ctrl Pts',(1.60896441674793,6.90553799888819,-5.69087246377536));
#168110=CARTESIAN_POINT('Ctrl Pts',(0.81436889005366,6.74169825447987,-5.85761036662907));
#168111=CARTESIAN_POINT('Ctrl Pts',(0.405257005850959,6.7,-5.9));
#168112=CARTESIAN_POINT('Ctrl Pts',(-0.40525700585096,6.7,-5.9));
#168113=CARTESIAN_POINT('Ctrl Pts',(-0.814368890053663,6.74169825447987,
-5.85761036662907));
#168114=CARTESIAN_POINT('Ctrl Pts',(-1.60896441674793,6.9055379988882,-5.69087246377536));
#168115=CARTESIAN_POINT('Ctrl Pts',(-1.99447655600236,7.02761131950198,
-5.56659302751097));
#168116=CARTESIAN_POINT('Ctrl Pts',(-2.69989199149733,7.32869287187661,
-5.25945052833492));
#168117=CARTESIAN_POINT('Ctrl Pts',(-3.02283773812843,7.50512371587152,
-5.07923593153682));
#168118=CARTESIAN_POINT('Ctrl Pts',(-3.31662479068874,7.70000000022112,
-4.87954915927577));
#168119=CARTESIAN_POINT('',(-3.96862696539036,8.19999999978668,-3.66196668634223));
#168120=CARTESIAN_POINT('Ctrl Pts',(-3.31662479061361,7.70000000017128,
-4.87954915911973));
#168121=CARTESIAN_POINT('Ctrl Pts',(-3.45417031520138,7.79123737951156,
-4.67574192153527));
#168122=CARTESIAN_POINT('Ctrl Pts',(-3.57693048224706,7.88087036673549,
-4.46762441021359));
#168123=CARTESIAN_POINT('Ctrl Pts',(-3.78526630624945,8.04294279611343,
-4.07348751507535));
#168124=CARTESIAN_POINT('Ctrl Pts',(-3.880589771382,8.1223584918038,-3.87186781082631));
#168125=CARTESIAN_POINT('Ctrl Pts',(-3.96862696589172,8.19999999937811,
-3.66196668640138));
#168126=CARTESIAN_POINT('',(-3.96862696466762,8.2,3.705910285));
#168127=CARTESIAN_POINT('Origin',(6.07153216583313E-15,12.7,-3.00000000000001));
#168128=CARTESIAN_POINT('',(3.96862696634616,8.19999999999999,-3.66196668499183));
#168129=CARTESIAN_POINT('',(3.96862696609543,8.19999999955775,-5.923067887));
#168130=CARTESIAN_POINT('Ctrl Pts',(3.96862696647649,8.19999999989382,-3.66196668500722));
#168131=CARTESIAN_POINT('Ctrl Pts',(3.88058977180391,8.12235849215553,-3.87186780993351));
#168132=CARTESIAN_POINT('Ctrl Pts',(3.78526630647339,8.04294279628764,-4.07348751465177));
#168133=CARTESIAN_POINT('Ctrl Pts',(3.57693048230356,7.88087036677944,-4.46762441010679));
#168134=CARTESIAN_POINT('Ctrl Pts',(3.45417031533094,7.79123737960611,-4.67574192131607));
#168135=CARTESIAN_POINT('Ctrl Pts',(3.31662479083111,7.70000000031555,-4.87954915879754));
#168136=CARTESIAN_POINT('Origin',(0.,5.2,-3.61270805748469E-16));
#168137=CARTESIAN_POINT('',(-7.22541611496938E-16,5.2,5.9));
#168138=CARTESIAN_POINT('',(-7.22541611496938E-16,5.2,5.9));
#168139=CARTESIAN_POINT('Origin',(0.,5.2,-1.28008620615991E-15));
#168140=CARTESIAN_POINT('Origin',(-1.99493199737333E-14,8.20000000000005,
-1.07349914972576E-14));
#168141=CARTESIAN_POINT('',(3.96862696634616,8.19999999977888,3.6619666853179));
#168142=CARTESIAN_POINT('Origin',(1.73472347597681E-14,8.19999999999999,
-2.12531425647619E-14));
#168143=CARTESIAN_POINT('',(3.31662479023432,7.69999999991968,4.87954915968175));
#168144=CARTESIAN_POINT('Ctrl Pts',(3.31662479023432,7.69999999991968,4.87954915968175));
#168145=CARTESIAN_POINT('Ctrl Pts',(3.53703437758293,7.84620318019848,4.55295860532687));
#168146=CARTESIAN_POINT('Ctrl Pts',(3.72403639169807,7.99140810117883,4.20771033743069));
#168147=CARTESIAN_POINT('Ctrl Pts',(3.90713471909885,8.14631670002404,3.8055381686148));
#168148=CARTESIAN_POINT('Ctrl Pts',(3.93825718793793,8.17321637276845,3.73437529255024));
#168149=CARTESIAN_POINT('Ctrl Pts',(3.96862696634616,8.19999999977888,3.66196668531789));
#168150=CARTESIAN_POINT('Origin',(0.,7.7,3.61270805748469E-16));
#168151=CARTESIAN_POINT('Origin',(0.,7.7,3.61270805748469E-16));
#168152=CARTESIAN_POINT('',(-4.90205800726441E-17,6.7,5.9));
#168153=CARTESIAN_POINT('',(-7.22541611496938E-16,7.7,5.9));
#168154=CARTESIAN_POINT('',(-3.3166247905171,7.70000000010726,4.87954915939243));
#168155=CARTESIAN_POINT('Ctrl Pts',(6.93889390390723E-16,6.7,5.9));
#168156=CARTESIAN_POINT('Ctrl Pts',(-0.405257005850958,6.7,5.9));
#168157=CARTESIAN_POINT('Ctrl Pts',(-0.81436889005366,6.74169825447987,
5.85761036662908));
#168158=CARTESIAN_POINT('Ctrl Pts',(-1.60896441674793,6.9055379988882,5.69087246377536));
#168159=CARTESIAN_POINT('Ctrl Pts',(-1.99447655600236,7.02761131950198,
5.56659302751097));
#168160=CARTESIAN_POINT('Ctrl Pts',(-2.69989199143067,7.32869287184816,
5.25945052836394));
#168161=CARTESIAN_POINT('Ctrl Pts',(-3.02283773800358,7.50512371580314,
5.07923593160667));
#168162=CARTESIAN_POINT('Ctrl Pts',(-3.3166247905182,7.700000000108,4.87954915939168));
#168163=CARTESIAN_POINT('Origin',(3.33197214177239E-15,7.70000000000001,
2.60208521393186E-15));
#168164=CARTESIAN_POINT('Ctrl Pts',(3.31662479020071,7.69999999989739,4.87954915960748));
#168165=CARTESIAN_POINT('Ctrl Pts',(3.02283773777115,7.50512371567581,5.07923593173671));
#168166=CARTESIAN_POINT('Ctrl Pts',(2.69989199130658,7.32869287179519,5.25945052841797));
#168167=CARTESIAN_POINT('Ctrl Pts',(1.99447655600236,7.02761131950198,5.56659302751097));
#168168=CARTESIAN_POINT('Ctrl Pts',(1.60896441674793,6.90553799888819,5.69087246377536));
#168169=CARTESIAN_POINT('Ctrl Pts',(0.814368890053661,6.74169825447987,
5.85761036662908));
#168170=CARTESIAN_POINT('Ctrl Pts',(0.405257005850959,6.7,5.9));
#168171=CARTESIAN_POINT('Ctrl Pts',(6.24500451351651E-16,6.7,5.9));
#168172=CARTESIAN_POINT('Origin',(-7.084,1.2,7.084));
#168173=CARTESIAN_POINT('Origin',(-7.084,1.7,7.084));
#168174=CARTESIAN_POINT('Origin',(3.354101966,3.2,3.));
#168175=CARTESIAN_POINT('Origin',(3.03576608295941E-15,12.7,3.));
#168176=CARTESIAN_POINT('',(3.354101966,3.2,3.));
#168177=CARTESIAN_POINT('Origin',(3.03576608295941E-15,12.7,2.098645905));
#168178=CARTESIAN_POINT('',(-3.96862696596741,8.19999999960437,3.66196668531925));
#168179=CARTESIAN_POINT('',(-3.96862696551168,8.19999999904294,2.098645905));
#168180=CARTESIAN_POINT('Ctrl Pts',(-3.96862696627435,8.19999999971555,
3.66196668548911));
#168181=CARTESIAN_POINT('Ctrl Pts',(-3.88058977165807,8.12235849203395,
3.87186781024209));
#168182=CARTESIAN_POINT('Ctrl Pts',(-3.78526630639598,8.04294279622742,
4.07348751479814));
#168183=CARTESIAN_POINT('Ctrl Pts',(-3.57693048220827,7.88087036670531,
4.467624410287));
#168184=CARTESIAN_POINT('Ctrl Pts',(-3.45417031511241,7.79123737944662,
4.67574192168587));
#168185=CARTESIAN_POINT('Ctrl Pts',(-3.31662479046424,7.7000000000722,4.87954915934106));
#168186=CARTESIAN_POINT('',(3.96862696609543,8.19999999955776,2.098645905));
#168187=CARTESIAN_POINT('Origin',(-5.408588238,8.2,3.705910285));
#168188=CARTESIAN_POINT('Origin',(2.60208521396521E-15,8.20000000000001,
2.60208521396521E-15));
#168189=CARTESIAN_POINT('Origin',(-3.354101966,3.2,-3.));
#168190=CARTESIAN_POINT('',(-3.354101966,3.2,-3.));
#168191=CARTESIAN_POINT('Origin',(-3.39435119,3.2,-4.509));
#168192=CARTESIAN_POINT('Origin',(-3.39435119,3.2,3.));
#168193=CARTESIAN_POINT('Origin',(3.968626967,8.2,3.705910285));
#168194=CARTESIAN_POINT('Origin',(2.60208521396521E-15,8.20000000000001,
2.60208521396521E-15));
#168195=CARTESIAN_POINT('Origin',(-1.06251812903579E-14,12.7,3.));
#168196=CARTESIAN_POINT('',(3.35410196856641,7.72506281602885,3.));
#168197=CARTESIAN_POINT('',(-3.3541019674191,7.72506281525532,3.));
#168198=CARTESIAN_POINT('Origin',(-1.06251812903579E-14,12.7,3.));
#168199=CARTESIAN_POINT('',(-1.78706256720332E-9,6.7,4.49999994459035));
#168200=CARTESIAN_POINT('Ctrl Pts',(-1.78706256720332E-9,6.7,4.49999994459035));
#168201=CARTESIAN_POINT('Ctrl Pts',(0.129339864826736,6.69999999996148,
4.50000046715268));
#168202=CARTESIAN_POINT('Ctrl Pts',(0.257887038991172,6.70417800065084,
4.4945561472941));
#168203=CARTESIAN_POINT('Ctrl Pts',(0.385634752023517,6.71240567188861,
4.48366782762931));
#168204=CARTESIAN_POINT('Ctrl Pts',(0.514978836758675,6.72073615844284,
4.47264344442968));
#168205=CARTESIAN_POINT('Ctrl Pts',(0.643504005298411,6.73321809239324,
4.45603815176915));
#168206=CARTESIAN_POINT('Ctrl Pts',(0.771213641489143,6.74977063306119,
4.43385282424746));
#168207=CARTESIAN_POINT('Ctrl Pts',(0.834706337055075,6.75799996842555,
4.42282306730522));
#168208=CARTESIAN_POINT('Ctrl Pts',(0.897997554075187,6.76723625943253,
4.41041407905336));
#168209=CARTESIAN_POINT('Ctrl Pts',(0.961087886286797,6.77747435000635,
4.39662596696742));
#168210=CARTESIAN_POINT('Ctrl Pts',(1.12537190708357,6.80413381788023,4.3607224233773));
#168211=CARTESIAN_POINT('Ctrl Pts',(1.28792473919659,6.83753175897511,4.31546645455455));
#168212=CARTESIAN_POINT('Ctrl Pts',(1.44821965309347,6.87740093803517,4.26085806049916));
#168213=CARTESIAN_POINT('Ctrl Pts',(1.59559285693051,6.91405617873864,4.21065176391313));
#168214=CARTESIAN_POINT('Ctrl Pts',(1.74105777043341,6.95618076529,4.15254010445229));
#168215=CARTESIAN_POINT('Ctrl Pts',(1.88423172912276,7.00353874840116,4.08652308211663));
#168216=CARTESIAN_POINT('Ctrl Pts',(1.90575246534007,7.01065721234285,4.07659994430202));
#168217=CARTESIAN_POINT('Ctrl Pts',(1.92586056099981,7.01743886839554,4.06714396610388));
#168218=CARTESIAN_POINT('Ctrl Pts',(1.94570126342584,7.0242404390687,4.05763019846389));
#168219=CARTESIAN_POINT('Ctrl Pts',(1.96030649260708,7.029247242575,4.05062688004424));
#168220=CARTESIAN_POINT('Ctrl Pts',(1.97476648543564,7.03426595278277,4.04359224671478));
#168221=CARTESIAN_POINT('Ctrl Pts',(1.98953237657893,7.03945577505624,4.03631690113625));
#168222=CARTESIAN_POINT('Ctrl Pts',(2.02435722390795,7.05169579271482,4.01915824836145));
#168223=CARTESIAN_POINT('Ctrl Pts',(2.05894905106974,7.064214991415,4.00155625212987));
#168224=CARTESIAN_POINT('Ctrl Pts',(2.09330430396177,7.07700461577505,3.98351091244152));
#168225=CARTESIAN_POINT('Ctrl Pts',(2.16201480974582,7.10258386449517,3.94742023306482));
#168226=CARTESIAN_POINT('Ctrl Pts',(2.22977900041436,7.12924486558745,3.90955617986103));
#168227=CARTESIAN_POINT('Ctrl Pts',(2.29657229433863,7.15691821304465,3.86991875283014));
#168228=CARTESIAN_POINT('Ctrl Pts',(2.43015888218718,7.21226490795906,3.79064389876838));
#168229=CARTESIAN_POINT('Ctrl Pts',(2.55985804007038,7.27166009599461,3.70427554939825));
#168230=CARTESIAN_POINT('Ctrl Pts',(2.68552125332657,7.3345572784782,3.61081370471976));
#168231=CARTESIAN_POINT('Ctrl Pts',(2.717569407263,7.35059807939496,3.58697793363111));
#168232=CARTESIAN_POINT('Ctrl Pts',(2.74838045933184,7.36637365233043,3.56343889776758));
#168233=CARTESIAN_POINT('Ctrl Pts',(2.77863399377477,7.38218154421955,3.53970081047817));
#168234=CARTESIAN_POINT('Ctrl Pts',(2.807693647199,7.39736561669651,3.51689948817693));
#168235=CARTESIAN_POINT('Ctrl Pts',(2.83623879778978,7.4125800305368,3.49391451461461));
#168236=CARTESIAN_POINT('Ctrl Pts',(2.86485150554233,7.42812880931336,3.47030651234304));
#168237=CARTESIAN_POINT('Ctrl Pts',(2.96506503774409,7.48258706108384,3.38762152788363));
#168238=CARTESIAN_POINT('Ctrl Pts',(3.06126197540171,7.53856247314563,3.30094146245984));
#168239=CARTESIAN_POINT('Ctrl Pts',(3.15352787595008,7.59556448413679,3.21026631607167));
#168240=CARTESIAN_POINT('Ctrl Pts',(3.22256997475172,7.63821879576605,3.14241457042591));
#168241=CARTESIAN_POINT('Ctrl Pts',(3.28941180762198,7.68144871837357,3.07232579840202));
#168242=CARTESIAN_POINT('Ctrl Pts',(3.35410196856641,7.72506281602885,3.));
#168243=CARTESIAN_POINT('Ctrl Pts',(-3.3541019674191,7.72506281525532,3.));
#168244=CARTESIAN_POINT('Ctrl Pts',(-3.26710242501228,7.66640773570053,
3.09726844444298));
#168245=CARTESIAN_POINT('Ctrl Pts',(-3.17621168160488,7.60844716360588,
3.19048950554114));
#168246=CARTESIAN_POINT('Ctrl Pts',(-3.08131599749725,7.55165155379247,
3.27966318329446));
#168247=CARTESIAN_POINT('Ctrl Pts',(-2.98857273444298,7.49614418029296,
3.36681422637049));
#168248=CARTESIAN_POINT('Ctrl Pts',(-2.89200380684714,7.44174972026469,
3.4500994090919));
#168249=CARTESIAN_POINT('Ctrl Pts',(-2.79153720797724,7.38894360635489,
3.52951873145868));
#168250=CARTESIAN_POINT('Ctrl Pts',(-2.75687850682911,7.37072669305851,
3.55691659891175));
#168251=CARTESIAN_POINT('Ctrl Pts',(-2.72175627382409,7.35269911657902,
3.5838543927489));
#168252=CARTESIAN_POINT('Ctrl Pts',(-2.68616864279695,7.33488135989013,
3.61033211297012));
#168253=CARTESIAN_POINT('Ctrl Pts',(-2.65488489637762,7.31921844089472,
3.63360767982455));
#168254=CARTESIAN_POINT('Ctrl Pts',(-2.62249728780483,7.30334972819107,
3.65704953038831));
#168255=CARTESIAN_POINT('Ctrl Pts',(-2.58964713218308,7.28763196643318,
3.68017390982419));
#168256=CARTESIAN_POINT('Ctrl Pts',(-2.55836408346407,7.27266401582474,
3.70219514761736));
#168257=CARTESIAN_POINT('Ctrl Pts',(-2.52666178411185,7.25783281963418,
3.72392848153279));
#168258=CARTESIAN_POINT('Ctrl Pts',(-2.49511365736935,7.24340693868336,
3.74495613869445));
#168259=CARTESIAN_POINT('Ctrl Pts',(-2.37311356381492,7.18762046235878,
3.82627241340996));
#168260=CARTESIAN_POINT('Ctrl Pts',(-2.24760162082057,7.13517639097339,
3.90130500603833));
#168261=CARTESIAN_POINT('Ctrl Pts',(-2.11872653965801,7.08653423897956,
3.97005391657957));
#168262=CARTESIAN_POINT('Ctrl Pts',(-2.04263766794184,7.05781552602381,
4.01064381951201));
#168263=CARTESIAN_POINT('Ctrl Pts',(-1.96537740734312,7.030422274254,4.0490433468627));
#168264=CARTESIAN_POINT('Ctrl Pts',(-1.88698486775426,7.00445014868043,
4.08525249863165));
#168265=CARTESIAN_POINT('Ctrl Pts',(-1.87314229568395,6.99986398497203,
4.09164631870172));
#168266=CARTESIAN_POINT('Ctrl Pts',(-1.85790374859226,6.99487575477689,
4.09859060754196));
#168267=CARTESIAN_POINT('Ctrl Pts',(-1.84288700566157,6.99002911703013,
4.10533727720876));
#168268=CARTESIAN_POINT('Ctrl Pts',(-1.83881362303491,6.98871443713673,
4.10716735228798));
#168269=CARTESIAN_POINT('Ctrl Pts',(-1.83475665416027,6.98740989272774,
4.10898288657729));
#168270=CARTESIAN_POINT('Ctrl Pts',(-1.83074859655393,6.98612569474828,
4.11076894900306));
#168271=CARTESIAN_POINT('Ctrl Pts',(-1.81196462019843,6.98010723222821,
4.11913942609453));
#168272=CARTESIAN_POINT('Ctrl Pts',(-1.7931423680753,6.97417864231932,4.1273748968128));
#168273=CARTESIAN_POINT('Ctrl Pts',(-1.77428267600905,6.96834046844946,
4.13547536115787));
#168274=CARTESIAN_POINT('Ctrl Pts',(-1.73656329187656,6.95666412070975,
4.15167628984802));
#168275=CARTESIAN_POINT('Ctrl Pts',(-1.69869414511969,6.94534944605757,
4.1673371930454));
#168276=CARTESIAN_POINT('Ctrl Pts',(-1.66068201913898,6.93440070493028,
4.18245807074999));
#168277=CARTESIAN_POINT('Ctrl Pts',(-1.58465776717757,6.9125032226757,4.21269982615919));
#168278=CARTESIAN_POINT('Ctrl Pts',(-1.50806156814689,6.89206961886207,
4.24078147959728));
#168279=CARTESIAN_POINT('Ctrl Pts',(-1.43094874001203,6.87313242784273,
4.26670303106426));
#168280=CARTESIAN_POINT('Ctrl Pts',(-1.27672308374233,6.83525804580405,
4.31854613399822));
#168281=CARTESIAN_POINT('Ctrl Pts',(-1.12043027200512,6.80337178019105,
4.36174882904776));
#168282=CARTESIAN_POINT('Ctrl Pts',(-0.962538453685088,6.77770992561345,
4.39631111621286));
#168283=CARTESIAN_POINT('Ctrl Pts',(-0.800364978502917,6.75135218155331,
4.43181065177745));
#168284=CARTESIAN_POINT('Ctrl Pts',(-0.636504623877591,6.73156143174531,
4.45819481027176));
#168285=CARTESIAN_POINT('Ctrl Pts',(-0.471495848535052,6.71855438336064,
4.47546359169579));
#168286=CARTESIAN_POINT('Ctrl Pts',(-0.315200100455022,6.70623415158282,
4.49182052244385));
#168287=CARTESIAN_POINT('Ctrl Pts',(-0.157874403365117,6.70000000004702,
4.49999930674204));
#168288=CARTESIAN_POINT('Ctrl Pts',(-1.78706256720332E-9,6.7,4.49999994459035));
#168289=CARTESIAN_POINT('Origin',(-1.06251812903579E-14,12.7,-4.50927590902132));
#168290=CARTESIAN_POINT('',(1.78651616390521E-9,6.7,-4.4999999445903));
#168291=CARTESIAN_POINT('',(-3.3541019674191,7.72506281525532,-3.));
#168292=CARTESIAN_POINT('Ctrl Pts',(1.78651616390521E-9,6.7,-4.4999999445903));
#168293=CARTESIAN_POINT('Ctrl Pts',(-0.1293400059774,6.69999999996149,-4.50000046715798));
#168294=CARTESIAN_POINT('Ctrl Pts',(-0.257887320736992,6.70417800978038,
-4.4945561354334));
#168295=CARTESIAN_POINT('Ctrl Pts',(-0.385635172884763,6.71240569899445,
-4.48366779203622));
#168296=CARTESIAN_POINT('Ctrl Pts',(-0.514979403716141,6.72073620408728,
-4.47264338436081));
#168297=CARTESIAN_POINT('Ctrl Pts',(-0.643504716769734,6.73321816598151,
-4.4560380546073));
#168298=CARTESIAN_POINT('Ctrl Pts',(-0.771214494975836,6.7497707436823,
-4.43385267738071));
#168299=CARTESIAN_POINT('Ctrl Pts',(-0.834706907564031,6.75800005162989,
-4.42282295715034));
#168300=CARTESIAN_POINT('Ctrl Pts',(-0.897997843233306,6.76723630625431,
-4.41041401785453));
#168301=CARTESIAN_POINT('Ctrl Pts',(-0.961087895601655,6.77747435151793,
-4.39662596696768));
#168302=CARTESIAN_POINT('Ctrl Pts',(-1.12537190818166,6.80413381832361,
-4.36072242527897));
#168303=CARTESIAN_POINT('Ctrl Pts',(-1.28792473154021,6.83753175756272,
-4.31546645934819));
#168304=CARTESIAN_POINT('Ctrl Pts',(-1.44821963626535,6.87740093384961,
-4.26085806917535));
#168305=CARTESIAN_POINT('Ctrl Pts',(-1.59559284796386,6.91405617605614,
-4.21065177060798));
#168306=CARTESIAN_POINT('Ctrl Pts',(-1.74105776855341,6.95618076454506,
-4.15254010825504));
#168307=CARTESIAN_POINT('Ctrl Pts',(-1.88423173353724,7.00353874986135,
-4.08652308211651));
#168308=CARTESIAN_POINT('Ctrl Pts',(-1.90575247663866,7.01065721609861,
-4.0765999409923));
#168309=CARTESIAN_POINT('Ctrl Pts',(-1.92586057997639,7.01743887479533,
-4.06714395901082));
#168310=CARTESIAN_POINT('Ctrl Pts',(-1.94570129044311,7.02424044833046,
-4.05763018730582));
#168311=CARTESIAN_POINT('Ctrl Pts',(-1.96030651405485,7.02924725000518,
-4.05062687140262));
#168312=CARTESIAN_POINT('Ctrl Pts',(-1.97476650173835,7.03426595848241,
-4.04359224048625));
#168313=CARTESIAN_POINT('Ctrl Pts',(-1.98953238692627,7.03945577869306,
-4.0363168977882));
#168314=CARTESIAN_POINT('Ctrl Pts',(-2.02435723598812,7.05169579703221,
-4.0191582440327));
#168315=CARTESIAN_POINT('Ctrl Pts',(-2.05894906457989,7.06421499634263,
-4.00155624698302));
#168316=CARTESIAN_POINT('Ctrl Pts',(-2.09330431860398,7.07700462122599,
-3.98351090663917));
#168317=CARTESIAN_POINT('Ctrl Pts',(-2.16201482665217,7.10258387099271,
-3.94742022595146));
#168318=CARTESIAN_POINT('Ctrl Pts',(-2.2297790183933,7.12924487278354,-3.90955617208706));
#168319=CARTESIAN_POINT('Ctrl Pts',(-2.29657231224609,7.15691822046394,
-3.86991874504595));
#168320=CARTESIAN_POINT('Ctrl Pts',(-2.43015889995167,7.21226491582476,
-3.79064389096373));
#168321=CARTESIAN_POINT('Ctrl Pts',(-2.55985805310911,7.27166010239785,
-3.7042755441747));
#168322=CARTESIAN_POINT('Ctrl Pts',(-2.68552125752396,7.33455728057908,
-3.61081370467886));
#168323=CARTESIAN_POINT('Ctrl Pts',(-2.71756942591652,7.3505980887628,-3.5869779224832));
#168324=CARTESIAN_POINT('Ctrl Pts',(-2.74838049300034,7.36637366956853,
-3.56343887448938));
#168325=CARTESIAN_POINT('Ctrl Pts',(-2.7786340426751,7.38218156977065,-3.53970077428726));
#168326=CARTESIAN_POINT('Ctrl Pts',(-2.80769367980225,7.39736563407233,
-3.51689946385006));
#168327=CARTESIAN_POINT('Ctrl Pts',(-2.83623881538779,7.41258004008775,
-3.4939145018208));
#168328=CARTESIAN_POINT('Ctrl Pts',(-2.86485150727639,7.42812881025568,
-3.47030651236767));
#168329=CARTESIAN_POINT('Ctrl Pts',(-2.96506504253387,7.4825870637294,-3.38762152443886));
#168330=CARTESIAN_POINT('Ctrl Pts',(-3.06126198327615,7.5385624777365,-3.30094145520137));
#168331=CARTESIAN_POINT('Ctrl Pts',(-3.1535278869199,7.59556449091396,-3.21026630465519));
#168332=CARTESIAN_POINT('Ctrl Pts',(-3.22256998125089,7.63821879998625,
-3.14241456256791));
#168333=CARTESIAN_POINT('Ctrl Pts',(-3.28941181008927,7.68144872005871,
-3.07232579434951));
#168334=CARTESIAN_POINT('Ctrl Pts',(-3.3541019674191,7.72506281525532,-3.));
#168335=CARTESIAN_POINT('',(3.35410196856641,7.72506281602885,-3.));
#168336=CARTESIAN_POINT('Ctrl Pts',(3.35410196856641,7.72506281602885,-3.));
#168337=CARTESIAN_POINT('Ctrl Pts',(3.26710242611272,7.66640773641328,-3.09726844451049));
#168338=CARTESIAN_POINT('Ctrl Pts',(3.17621168265789,7.60844716426129,-3.19048950566652));
#168339=CARTESIAN_POINT('Ctrl Pts',(3.08131599850246,7.55165155439411,-3.27966318346809));
#168340=CARTESIAN_POINT('Ctrl Pts',(2.98857273540257,7.49614418084271,-3.36681422659025));
#168341=CARTESIAN_POINT('Ctrl Pts',(2.89200380776084,7.44174972076591,-3.45009940934867));
#168342=CARTESIAN_POINT('Ctrl Pts',(2.79153720884502,7.38894360681101,-3.52951873174336));
#168343=CARTESIAN_POINT('Ctrl Pts',(2.75687850781638,7.37072669357022,-3.55691659909906));
#168344=CARTESIAN_POINT('Ctrl Pts',(2.72175627493448,7.35269911714525,-3.58385439284135));
#168345=CARTESIAN_POINT('Ctrl Pts',(2.68616864403411,7.33488136050956,-3.61033211297022));
#168346=CARTESIAN_POINT('Ctrl Pts',(2.65488489768749,7.31921844154152,-3.63360767977228));
#168347=CARTESIAN_POINT('Ctrl Pts',(2.62249728918549,7.30334972886251,-3.657049530288));
#168348=CARTESIAN_POINT('Ctrl Pts',(2.58964713363384,7.28763196712734,-3.68017390967919));
#168349=CARTESIAN_POINT('Ctrl Pts',(2.55836408484669,7.27266401647599,-3.70219514752476));
#168350=CARTESIAN_POINT('Ctrl Pts',(2.52666178542208,7.25783282024199,-3.72392848149313));
#168351=CARTESIAN_POINT('Ctrl Pts',(2.49511365861142,7.24340693925133,-3.74495613870205));
#168352=CARTESIAN_POINT('Ctrl Pts',(2.37311356491555,7.18762046282849,-3.82627241351892));
#168353=CARTESIAN_POINT('Ctrl Pts',(2.24760162177669,7.13517639135551,-3.90130500623051));
#168354=CARTESIAN_POINT('Ctrl Pts',(2.11872654046758,7.08653423928513,-3.97005391683681));
#168355=CARTESIAN_POINT('Ctrl Pts',(2.04263766891244,7.05781552637762,-4.01064381967561));
#168356=CARTESIAN_POINT('Ctrl Pts',(1.96537740848167,7.03042227465128,-4.04904334694059));
#168357=CARTESIAN_POINT('Ctrl Pts',(1.8869848690675,7.00445014911552,-4.08525249863175));
#168358=CARTESIAN_POINT('Ctrl Pts',(1.87314229700001,6.99986398540452,-4.09164631870103));
#168359=CARTESIAN_POINT('Ctrl Pts',(1.85790374991078,6.99487575520629,-4.09859060754057));
#168360=CARTESIAN_POINT('Ctrl Pts',(1.84288700698222,6.99002911745638,-4.10533727720669));
#168361=CARTESIAN_POINT('Ctrl Pts',(1.83881362435573,6.98871443756199,-4.10716735228591));
#168362=CARTESIAN_POINT('Ctrl Pts',(1.83475665548124,6.98740989315202,-4.10898288657522));
#168363=CARTESIAN_POINT('Ctrl Pts',(1.83074859787505,6.98612569517158,-4.11076894900098));
#168364=CARTESIAN_POINT('Ctrl Pts',(1.81196462152168,6.98010723264741,-4.11913942609173));
#168365=CARTESIAN_POINT('Ctrl Pts',(1.79314236940019,6.97417864273424,-4.12737489680932));
#168366=CARTESIAN_POINT('Ctrl Pts',(1.77428267733507,6.96834046885995,-4.13547536115374));
#168367=CARTESIAN_POINT('Ctrl Pts',(1.73656329320483,6.95666412111137,-4.15167628984257));
#168368=CARTESIAN_POINT('Ctrl Pts',(1.69869414644819,6.9453494464497,-4.16733719303872));
#168369=CARTESIAN_POINT('Ctrl Pts',(1.66068202046566,6.93440070531241,-4.18245807074219));
#168370=CARTESIAN_POINT('Ctrl Pts',(1.5846577685006,6.91250322303784,-4.21269982614912));
#168371=CARTESIAN_POINT('Ctrl Pts',(1.50806156945806,6.89206961920218,-4.24078147958532));
#168372=CARTESIAN_POINT('Ctrl Pts',(1.43094874130287,6.87313242815974,-4.26670303105079));
#168373=CARTESIAN_POINT('Ctrl Pts',(1.27672308499251,6.83525804607485,-4.31854613398173));
#168374=CARTESIAN_POINT('Ctrl Pts',(1.12043027318078,6.80337178041132,-4.36174882902975));
#168375=CARTESIAN_POINT('Ctrl Pts',(0.96253845475154,6.77770992578678,-4.39631111619484));
#168376=CARTESIAN_POINT('Ctrl Pts',(0.800364980059648,6.75135218177635,
-4.43181065162754));
#168377=CARTESIAN_POINT('Ctrl Pts',(0.636504625900533,6.73156143197304,
-4.45819481005927));
#168378=CARTESIAN_POINT('Ctrl Pts',(0.471495850994567,6.71855438355452,
-4.47546359149004));
#168379=CARTESIAN_POINT('Ctrl Pts',(0.315200102134448,6.70623415165054,
-4.4918205223694));
#168380=CARTESIAN_POINT('Ctrl Pts',(0.157874404222107,6.70000000004701,
-4.49999930673615));
#168381=CARTESIAN_POINT('Ctrl Pts',(1.78651616390521E-9,6.7,-4.4999999445903));
#168382=CARTESIAN_POINT('Origin',(-1.06251812903579E-14,12.7,-3.));
#170237=UNCERTAINTY_MEASURE_WITH_UNIT(LENGTH_MEASURE(0.01),#170251,
'DISTANCE_ACCURACY_VALUE',
'Maximum model space distance between geometric entities at asserted c
onnectivities');
#170242=UNCERTAINTY_MEASURE_WITH_UNIT(LENGTH_MEASURE(0.01),#170251,
'DISTANCE_ACCURACY_VALUE',
'Maximum model space distance between geometric entities at asserted c
onnectivities');
#170245=(
GEOMETRIC_REPRESENTATION_CONTEXT(3)
GLOBAL_UNCERTAINTY_ASSIGNED_CONTEXT((#170237))
GLOBAL_UNIT_ASSIGNED_CONTEXT((#170251,#170253,#170254))
REPRESENTATION_CONTEXT('','3D')
);
#170250=(
GEOMETRIC_REPRESENTATION_CONTEXT(3)
GLOBAL_UNCERTAINTY_ASSIGNED_CONTEXT((#170242))
GLOBAL_UNIT_ASSIGNED_CONTEXT((#170251,#170253,#170254))
REPRESENTATION_CONTEXT('','3D')
);
#170251=(
LENGTH_UNIT()
NAMED_UNIT(*)
SI_UNIT(.MILLI.,.METRE.)
);
#170253=(
NAMED_UNIT(*)
PLANE_ANGLE_UNIT()
SI_UNIT($,.RADIAN.)
);
#170254=(
NAMED_UNIT(*)
SI_UNIT($,.STERADIAN.)
SOLID_ANGLE_UNIT()
);
#170257=SHAPE_DEFINITION_REPRESENTATION(#170264,#170277);
#170264=PRODUCT_DEFINITION_SHAPE('',$,#170285);
#170277=SHAPE_REPRESENTATION('',(#77641,#42,#43),#170245);
#170282=PRODUCT_DEFINITION_CONTEXT('part definition',#170305,'design');
#170285=PRODUCT_DEFINITION('2026-11-14-09-55-10-334_1','Plunger base',#170292,
#170282);
#170292=PRODUCT_DEFINITION_FORMATION('',$,#170309);
#170305=APPLICATION_CONTEXT(
'Core Data for Automotive Mechanical Design Process');
#170306=PRODUCT_CONTEXT('part definition',#170305,'mechanical');
#170309=PRODUCT('2026-11-14-09-55-10-334_1','Plunger base',$,(#170306));
#170314=PRESENTATION_STYLE_ASSIGNMENT((#170318));
#170318=SURFACE_STYLE_USAGE(.BOTH.,#170322);
#170322=SURFACE_SIDE_STYLE('',(#170326));
#170326=SURFACE_STYLE_FILL_AREA(#170330);
#170330=FILL_AREA_STYLE('Steel - Satin',(#170334));
#170334=FILL_AREA_STYLE_COLOUR('Steel - Satin',#170338);
#170338=COLOUR_RGB('Steel - Satin',0.627450980392157,0.627450980392157,
0.627450980392157);
ENDSEC;
END-ISO-10303-21;
